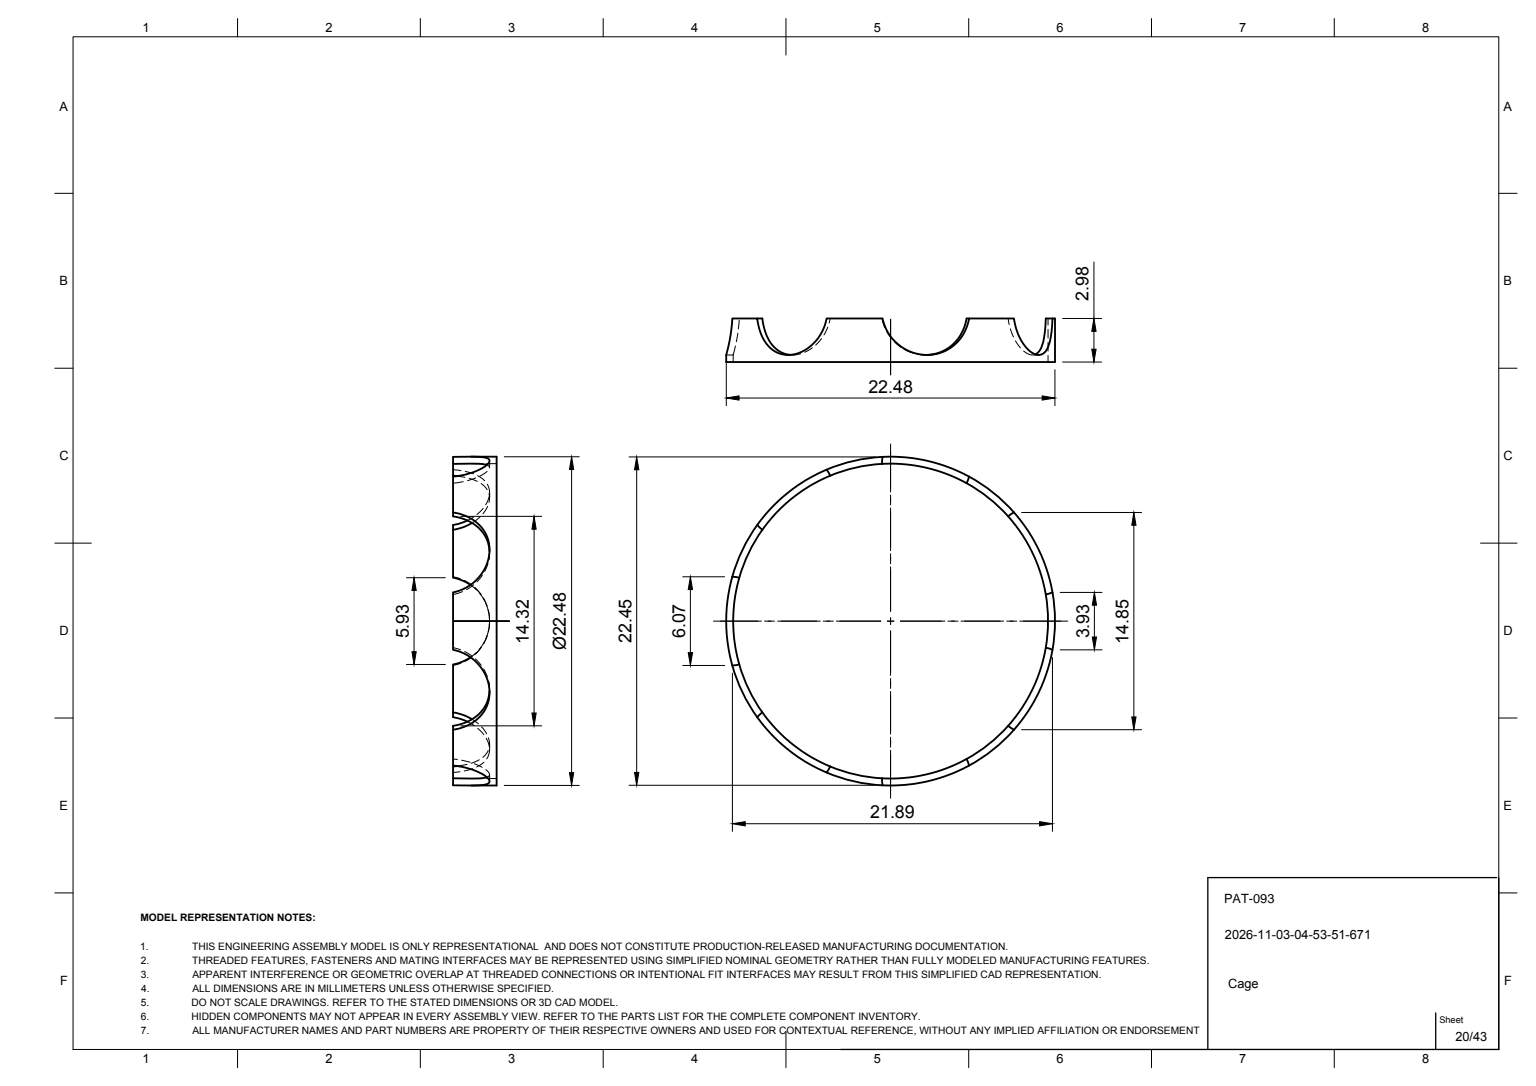
ISO-10303-21;
HEADER;
/* Generated by software containing ST-Developer
 * from STEP Tools, Inc. (www.steptools.com) 
 */

FILE_DESCRIPTION(
/* description */ ('Self-centering screw clamp'),
/* implementation_level */ '2;1');

FILE_NAME(
/* name */ 'Cage.step',
/* time_stamp */ '2026-10-28T03:25:31-07:00',
/* author */ (''),
/* organization */ (''),
/* preprocessor_version */ 'ST-DEVELOPER v20.2',
/* originating_system */ 'Autodesk Translation Framework v15.17.0.0',
/* authorisation */ '');

FILE_SCHEMA (('AUTOMOTIVE_DESIGN { 1 0 10303 214 3 1 1 }'));
ENDSEC;

DATA;
#10=MECHANICAL_DESIGN_GEOMETRIC_PRESENTATION_REPRESENTATION('',(#647),#16799);
#474=SPHERICAL_SURFACE('',#10011,0.309556);
#475=SPHERICAL_SURFACE('',#10027,0.309556);
#476=SPHERICAL_SURFACE('',#10032,0.309556);
#477=SPHERICAL_SURFACE('',#10038,0.309556);
#478=SPHERICAL_SURFACE('',#10043,0.309556);
#479=SPHERICAL_SURFACE('',#10048,0.309556);
#480=SPHERICAL_SURFACE('',#10056,0.309556);
#514=B_SPLINE_CURVE_WITH_KNOTS('',3,(#14785,#14786,#14787,#14788,#14789,
#14790,#14791,#14792,#14793,#14794,#14795,#14796,#14797,#14798,#14799,#14800,
#14801,#14802,#14803,#14804,#14805,#14806),.UNSPECIFIED.,.F.,.F.,(4,2,2,
2,2,2,2,2,2,2,4),(0.0591825211272536,0.157966726598481,0.236950089897721,
0.315933453196962,0.391576304923761,0.46721915665056,0.54286200837736,0.618504860104159,
0.697488223403399,0.77647158670264,0.875255792173867),.UNSPECIFIED.);
#515=B_SPLINE_CURVE_WITH_KNOTS('',3,(#14810,#14811,#14812,#14813,#14814,
#14815,#14816,#14817,#14818,#14819,#14820,#14821,#14822,#14823,#14824,#14825,
#14826,#14827,#14828,#14829,#14830,#14831),.UNSPECIFIED.,.F.,.F.,(4,2,2,
2,2,2,2,2,2,2,4),(0.0581119756758434,0.106553146291161,0.213106292582322,
0.30849933801665,0.386091982889075,0.4636846277615,0.541277272633925,0.61886991750635,
0.714262962940678,0.820816109231839,0.869257279847157),.UNSPECIFIED.);
#516=B_SPLINE_CURVE_WITH_KNOTS('',3,(#14837,#14838,#14839,#14840,#14841,
#14842,#14843,#14844,#14845,#14846,#14847,#14848,#14849,#14850,#14851,#14852,
#14853,#14854,#14855,#14856,#14857,#14858),.UNSPECIFIED.,.F.,.F.,(4,2,2,
2,2,2,2,2,2,2,4),(0.0581119756758434,0.106553146291161,0.213106292582322,
0.30849933801665,0.386091982889075,0.4636846277615,0.541277272633925,0.61886991750635,
0.714262962940679,0.820816109231839,0.869257279847157),.UNSPECIFIED.);
#517=B_SPLINE_CURVE_WITH_KNOTS('',3,(#14862,#14863,#14864,#14865,#14866,
#14867,#14868,#14869,#14870,#14871,#14872,#14873,#14874,#14875,#14876,#14877,
#14878,#14879,#14880,#14881,#14882,#14883),.UNSPECIFIED.,.F.,.F.,(4,2,2,
2,2,2,2,2,2,2,4),(0.0581119756758433,0.106553146291161,0.213106292582322,
0.308499338016649,0.386091982889075,0.4636846277615,0.541277272633925,0.61886991750635,
0.714262962940678,0.820816109231839,0.869257279847157),.UNSPECIFIED.);
#518=B_SPLINE_CURVE_WITH_KNOTS('',3,(#14892,#14893,#14894,#14895,#14896,
#14897,#14898,#14899,#14900,#14901,#14902,#14903,#14904,#14905,#14906,#14907,
#14908,#14909,#14910,#14911,#14912,#14913),.UNSPECIFIED.,.F.,.F.,(4,2,2,
2,2,2,2,2,2,2,4),(0.0581119756758433,0.106553146291161,0.213106292582322,
0.30849933801665,0.386091982889075,0.4636846277615,0.541277272633925,0.61886991750635,
0.714262962940678,0.820816109231839,0.869257279847157),.UNSPECIFIED.);
#519=B_SPLINE_CURVE_WITH_KNOTS('',3,(#14917,#14918,#14919,#14920,#14921,
#14922,#14923,#14924,#14925,#14926,#14927,#14928,#14929,#14930,#14931,#14932,
#14933,#14934,#14935,#14936,#14937,#14938),.UNSPECIFIED.,.F.,.F.,(4,2,2,
2,2,2,2,2,2,2,4),(0.0581119756758434,0.106553146291161,0.213106292582322,
0.30849933801665,0.386091982889075,0.4636846277615,0.541277272633925,0.61886991750635,
0.714262962940678,0.820816109231839,0.869257279847157),.UNSPECIFIED.);
#520=B_SPLINE_CURVE_WITH_KNOTS('',3,(#14942,#14943,#14944,#14945,#14946,
#14947,#14948,#14949,#14950,#14951,#14952,#14953,#14954,#14955,#14956,#14957,
#14958,#14959,#14960,#14961,#14962,#14963),.UNSPECIFIED.,.F.,.F.,(4,2,2,
2,2,2,2,2,2,2,4),(0.0581119756758434,0.106553146291161,0.213106292582322,
0.30849933801665,0.386091982889075,0.4636846277615,0.541277272633925,0.61886991750635,
0.714262962940678,0.820816109231839,0.869257279847157),.UNSPECIFIED.);
#521=B_SPLINE_CURVE_WITH_KNOTS('',3,(#14967,#14968,#14969,#14970,#14971,
#14972,#14973,#14974,#14975,#14976,#14977,#14978,#14979,#14980,#14981,#14982,
#14983,#14984,#14985,#14986,#14987,#14988),.UNSPECIFIED.,.F.,.F.,(4,2,2,
2,2,2,2,2,2,2,4),(0.0581119756758433,0.106553146291161,0.213106292582322,
0.30849933801665,0.386091982889075,0.4636846277615,0.541277272633925,0.61886991750635,
0.714262962940678,0.820816109231839,0.869257279847157),.UNSPECIFIED.);
#522=B_SPLINE_CURVE_WITH_KNOTS('',3,(#14996,#14997,#14998,#14999,#15000,
#15001,#15002,#15003,#15004,#15005,#15006,#15007,#15008,#15009,#15010,#15011,
#15012,#15013,#15014,#15015,#15016,#15017),.UNSPECIFIED.,.F.,.F.,(4,2,2,
2,2,2,2,2,2,2,4),(0.0591825211272536,0.157966726598481,0.236950089897721,
0.315933453196962,0.391576304923761,0.467219156650561,0.54286200837736,
0.618504860104159,0.697488223403399,0.77647158670264,0.875255792173867),
 .UNSPECIFIED.);
#523=B_SPLINE_CURVE_WITH_KNOTS('',3,(#15025,#15026,#15027,#15028,#15029,
#15030,#15031,#15032,#15033,#15034,#15035,#15036,#15037,#15038,#15039,#15040,
#15041,#15042,#15043,#15044,#15045,#15046),.UNSPECIFIED.,.F.,.F.,(4,2,2,
2,2,2,2,2,2,2,4),(0.0591825211272536,0.157966726598481,0.236950089897722,
0.315933453196962,0.391576304923761,0.467219156650561,0.54286200837736,
0.618504860104159,0.697488223403399,0.77647158670264,0.875255792173867),
 .UNSPECIFIED.);
#524=B_SPLINE_CURVE_WITH_KNOTS('',3,(#15056,#15057,#15058,#15059,#15060,
#15061,#15062,#15063,#15064,#15065,#15066,#15067,#15068,#15069,#15070,#15071,
#15072,#15073,#15074,#15075,#15076,#15077),.UNSPECIFIED.,.F.,.F.,(4,2,2,
2,2,2,2,2,2,2,4),(0.0591825211272536,0.157966726598481,0.236950089897721,
0.315933453196962,0.391576304923761,0.46721915665056,0.54286200837736,0.618504860104159,
0.697488223403399,0.77647158670264,0.875255792173867),.UNSPECIFIED.);
#525=B_SPLINE_CURVE_WITH_KNOTS('',3,(#15085,#15086,#15087,#15088,#15089,
#15090,#15091,#15092,#15093,#15094,#15095,#15096,#15097,#15098,#15099,#15100,
#15101,#15102,#15103,#15104,#15105,#15106),.UNSPECIFIED.,.F.,.F.,(4,2,2,
2,2,2,2,2,2,2,4),(0.0591825211272536,0.157966726598481,0.236950089897721,
0.315933453196962,0.391576304923761,0.46721915665056,0.542862008377359,
0.618504860104159,0.697488223403399,0.776471586702639,0.875255792173867),
 .UNSPECIFIED.);
#526=B_SPLINE_CURVE_WITH_KNOTS('',3,(#15114,#15115,#15116,#15117,#15118,
#15119,#15120,#15121,#15122,#15123,#15124,#15125,#15126,#15127,#15128,#15129,
#15130,#15131,#15132,#15133,#15134,#15135),.UNSPECIFIED.,.F.,.F.,(4,2,2,
2,2,2,2,2,2,2,4),(0.0591825211272536,0.157966726598481,0.236950089897721,
0.315933453196962,0.391576304923761,0.46721915665056,0.54286200837736,0.618504860104159,
0.697488223403399,0.77647158670264,0.875255792173867),.UNSPECIFIED.);
#527=B_SPLINE_CURVE_WITH_KNOTS('',3,(#15144,#15145,#15146,#15147,#15148,
#15149,#15150,#15151,#15152,#15153,#15154,#15155,#15156,#15157,#15158,#15159,
#15160,#15161,#15162,#15163,#15164,#15165),.UNSPECIFIED.,.F.,.F.,(4,2,2,
2,2,2,2,2,2,2,4),(0.0591825211272536,0.157966726598481,0.236950089897721,
0.315933453196962,0.391576304923761,0.46721915665056,0.542862008377359,
0.618504860104159,0.697488223403399,0.776471586702639,0.875255792173867),
 .UNSPECIFIED.);
#559=SHAPE_REPRESENTATION_RELATIONSHIP('SRR','None',#17033,#600);
#600=ADVANCED_BREP_SHAPE_REPRESENTATION('',(#695),#16771);
#647=STYLED_ITEM('',(#17326),#695);
#695=MANIFOLD_SOLID_BREP('Continuous crown cage',#9098);
#846=FACE_BOUND('',#2125,.T.);
#1110=PLANE('',#10024);
#1111=PLANE('',#10029);
#1112=PLANE('',#10034);
#1113=PLANE('',#10040);
#1114=PLANE('',#10045);
#1115=PLANE('',#10054);
#1116=PLANE('',#10058);
#1117=PLANE('',#10059);
#1477=FACE_OUTER_BOUND('',#2109,.T.);
#1478=FACE_OUTER_BOUND('',#2110,.T.);
#1479=FACE_OUTER_BOUND('',#2111,.T.);
#1480=FACE_OUTER_BOUND('',#2112,.T.);
#1481=FACE_OUTER_BOUND('',#2113,.T.);
#1482=FACE_OUTER_BOUND('',#2114,.T.);
#1483=FACE_OUTER_BOUND('',#2115,.T.);
#1484=FACE_OUTER_BOUND('',#2116,.T.);
#1485=FACE_OUTER_BOUND('',#2117,.T.);
#1486=FACE_OUTER_BOUND('',#2118,.T.);
#1487=FACE_OUTER_BOUND('',#2119,.T.);
#1488=FACE_OUTER_BOUND('',#2120,.T.);
#1489=FACE_OUTER_BOUND('',#2121,.T.);
#1490=FACE_OUTER_BOUND('',#2122,.T.);
#1491=FACE_OUTER_BOUND('',#2123,.T.);
#1492=FACE_OUTER_BOUND('',#2124,.T.);
#1493=FACE_OUTER_BOUND('',#2126,.T.);
#2109=EDGE_LOOP('',(#7071,#7072,#7073,#7074));
#2110=EDGE_LOOP('',(#7075,#7076,#7077,#7078,#7079,#7080,#7081,#7082,#7083,
#7084,#7085,#7086,#7087,#7088,#7089,#7090,#7091,#7092));
#2111=EDGE_LOOP('',(#7093,#7094,#7095,#7096));
#2112=EDGE_LOOP('',(#7097,#7098,#7099,#7100));
#2113=EDGE_LOOP('',(#7101,#7102,#7103,#7104));
#2114=EDGE_LOOP('',(#7105,#7106,#7107,#7108));
#2115=EDGE_LOOP('',(#7109,#7110,#7111,#7112,#7113,#7114));
#2116=EDGE_LOOP('',(#7115,#7116,#7117,#7118));
#2117=EDGE_LOOP('',(#7119,#7120,#7121,#7122));
#2118=EDGE_LOOP('',(#7123,#7124,#7125,#7126));
#2119=EDGE_LOOP('',(#7127,#7128,#7129,#7130));
#2120=EDGE_LOOP('',(#7131,#7132,#7133,#7134));
#2121=EDGE_LOOP('',(#7135,#7136,#7137,#7138,#7139,#7140,#7141,#7142,#7143,
#7144,#7145,#7146,#7147,#7148,#7149,#7150,#7151,#7152));
#2122=EDGE_LOOP('',(#7153,#7154,#7155,#7156));
#2123=EDGE_LOOP('',(#7157,#7158,#7159,#7160));
#2124=EDGE_LOOP('',(#7161));
#2125=EDGE_LOOP('',(#7162));
#2126=EDGE_LOOP('',(#7163,#7164,#7165,#7166));
#2836=LINE('',#14887,#3409);
#2837=LINE('',#15140,#3410);
#3409=VECTOR('',#11893,1.123812);
#3410=VECTOR('',#11962,1.076188);
#3932=CIRCLE('',#10012,0.303778037777585);
#3933=CIRCLE('',#10013,0.303778037777585);
#3934=CIRCLE('',#10015,1.123812);
#3935=CIRCLE('',#10016,1.123812);
#3936=CIRCLE('',#10017,1.123812);
#3937=CIRCLE('',#10018,1.123812);
#3938=CIRCLE('',#10019,1.123812);
#3939=CIRCLE('',#10020,1.123812);
#3940=CIRCLE('',#10021,1.123812);
#3941=CIRCLE('',#10022,1.123812);
#3942=CIRCLE('',#10023,1.123812);
#3943=CIRCLE('',#10025,1.076188);
#3944=CIRCLE('',#10026,0.303778037777585);
#3945=CIRCLE('',#10028,0.303778037777585);
#3946=CIRCLE('',#10030,1.076188);
#3947=CIRCLE('',#10031,0.303778037777585);
#3948=CIRCLE('',#10033,0.303778037777585);
#3949=CIRCLE('',#10035,1.076188);
#3950=CIRCLE('',#10036,1.076188);
#3951=CIRCLE('',#10037,0.303778037777585);
#3952=CIRCLE('',#10039,0.303778037777585);
#3953=CIRCLE('',#10041,1.076188);
#3954=CIRCLE('',#10042,0.303778037777585);
#3955=CIRCLE('',#10044,0.303778037777585);
#3956=CIRCLE('',#10046,1.076188);
#3957=CIRCLE('',#10047,0.303778037777585);
#3958=CIRCLE('',#10049,0.303778037777585);
#3959=CIRCLE('',#10051,1.076188);
#3960=CIRCLE('',#10052,1.076188);
#3961=CIRCLE('',#10053,1.076188);
#3962=CIRCLE('',#10055,0.303778037777585);
#3963=CIRCLE('',#10057,0.303778037777585);
#4551=VERTEX_POINT('',#14783);
#4552=VERTEX_POINT('',#14784);
#4553=VERTEX_POINT('',#14807);
#4554=VERTEX_POINT('',#14809);
#4555=VERTEX_POINT('',#14834);
#4556=VERTEX_POINT('',#14836);
#4557=VERTEX_POINT('',#14859);
#4558=VERTEX_POINT('',#14861);
#4559=VERTEX_POINT('',#14884);
#4560=VERTEX_POINT('',#14886);
#4561=VERTEX_POINT('',#14889);
#4562=VERTEX_POINT('',#14891);
#4563=VERTEX_POINT('',#14914);
#4564=VERTEX_POINT('',#14916);
#4565=VERTEX_POINT('',#14939);
#4566=VERTEX_POINT('',#14941);
#4567=VERTEX_POINT('',#14964);
#4568=VERTEX_POINT('',#14966);
#4569=VERTEX_POINT('',#14991);
#4570=VERTEX_POINT('',#14995);
#4571=VERTEX_POINT('',#15020);
#4572=VERTEX_POINT('',#15024);
#4573=VERTEX_POINT('',#15049);
#4574=VERTEX_POINT('',#15051);
#4575=VERTEX_POINT('',#15055);
#4576=VERTEX_POINT('',#15080);
#4577=VERTEX_POINT('',#15084);
#4578=VERTEX_POINT('',#15109);
#4579=VERTEX_POINT('',#15113);
#4580=VERTEX_POINT('',#15138);
#4581=VERTEX_POINT('',#15141);
#4582=VERTEX_POINT('',#15143);
#5460=EDGE_CURVE('',#4551,#4552,#514,.T.);
#5461=EDGE_CURVE('',#4553,#4551,#3932,.T.);
#5462=EDGE_CURVE('',#4554,#4553,#515,.T.);
#5463=EDGE_CURVE('',#4552,#4554,#3933,.T.);
#5464=EDGE_CURVE('',#4555,#4553,#3934,.T.);
#5465=EDGE_CURVE('',#4555,#4556,#516,.T.);
#5466=EDGE_CURVE('',#4557,#4556,#3935,.T.);
#5467=EDGE_CURVE('',#4557,#4558,#517,.T.);
#5468=EDGE_CURVE('',#4559,#4558,#3936,.T.);
#5469=EDGE_CURVE('',#4559,#4560,#2836,.T.);
#5470=EDGE_CURVE('',#4560,#4560,#3937,.T.);
#5471=EDGE_CURVE('',#4561,#4559,#3938,.T.);
#5472=EDGE_CURVE('',#4561,#4562,#518,.T.);
#5473=EDGE_CURVE('',#4563,#4562,#3939,.T.);
#5474=EDGE_CURVE('',#4563,#4564,#519,.T.);
#5475=EDGE_CURVE('',#4565,#4564,#3940,.T.);
#5476=EDGE_CURVE('',#4565,#4566,#520,.T.);
#5477=EDGE_CURVE('',#4567,#4566,#3941,.T.);
#5478=EDGE_CURVE('',#4567,#4568,#521,.T.);
#5479=EDGE_CURVE('',#4554,#4568,#3942,.T.);
#5480=EDGE_CURVE('',#4551,#4569,#3943,.T.);
#5481=EDGE_CURVE('',#4569,#4555,#3944,.T.);
#5482=EDGE_CURVE('',#4570,#4569,#522,.T.);
#5483=EDGE_CURVE('',#4556,#4570,#3945,.T.);
#5484=EDGE_CURVE('',#4570,#4571,#3946,.T.);
#5485=EDGE_CURVE('',#4571,#4557,#3947,.T.);
#5486=EDGE_CURVE('',#4572,#4571,#523,.T.);
#5487=EDGE_CURVE('',#4558,#4572,#3948,.T.);
#5488=EDGE_CURVE('',#4572,#4573,#3949,.T.);
#5489=EDGE_CURVE('',#4573,#4574,#3950,.T.);
#5490=EDGE_CURVE('',#4574,#4561,#3951,.T.);
#5491=EDGE_CURVE('',#4575,#4574,#524,.T.);
#5492=EDGE_CURVE('',#4562,#4575,#3952,.T.);
#5493=EDGE_CURVE('',#4575,#4576,#3953,.T.);
#5494=EDGE_CURVE('',#4576,#4563,#3954,.T.);
#5495=EDGE_CURVE('',#4577,#4576,#525,.T.);
#5496=EDGE_CURVE('',#4564,#4577,#3955,.T.);
#5497=EDGE_CURVE('',#4577,#4578,#3956,.T.);
#5498=EDGE_CURVE('',#4578,#4565,#3957,.T.);
#5499=EDGE_CURVE('',#4579,#4578,#526,.T.);
#5500=EDGE_CURVE('',#4566,#4579,#3958,.T.);
#5501=EDGE_CURVE('',#4580,#4580,#3959,.T.);
#5502=EDGE_CURVE('',#4580,#4573,#2837,.T.);
#5503=EDGE_CURVE('',#4581,#4552,#3960,.T.);
#5504=EDGE_CURVE('',#4581,#4582,#527,.T.);
#5505=EDGE_CURVE('',#4579,#4582,#3961,.T.);
#5506=EDGE_CURVE('',#4568,#4581,#3962,.T.);
#5507=EDGE_CURVE('',#4582,#4567,#3963,.T.);
#7071=ORIENTED_EDGE('',*,*,#5460,.F.);
#7072=ORIENTED_EDGE('',*,*,#5461,.F.);
#7073=ORIENTED_EDGE('',*,*,#5462,.F.);
#7074=ORIENTED_EDGE('',*,*,#5463,.F.);
#7075=ORIENTED_EDGE('',*,*,#5462,.T.);
#7076=ORIENTED_EDGE('',*,*,#5464,.F.);
#7077=ORIENTED_EDGE('',*,*,#5465,.T.);
#7078=ORIENTED_EDGE('',*,*,#5466,.F.);
#7079=ORIENTED_EDGE('',*,*,#5467,.T.);
#7080=ORIENTED_EDGE('',*,*,#5468,.F.);
#7081=ORIENTED_EDGE('',*,*,#5469,.T.);
#7082=ORIENTED_EDGE('',*,*,#5470,.F.);
#7083=ORIENTED_EDGE('',*,*,#5469,.F.);
#7084=ORIENTED_EDGE('',*,*,#5471,.F.);
#7085=ORIENTED_EDGE('',*,*,#5472,.T.);
#7086=ORIENTED_EDGE('',*,*,#5473,.F.);
#7087=ORIENTED_EDGE('',*,*,#5474,.T.);
#7088=ORIENTED_EDGE('',*,*,#5475,.F.);
#7089=ORIENTED_EDGE('',*,*,#5476,.T.);
#7090=ORIENTED_EDGE('',*,*,#5477,.F.);
#7091=ORIENTED_EDGE('',*,*,#5478,.T.);
#7092=ORIENTED_EDGE('',*,*,#5479,.F.);
#7093=ORIENTED_EDGE('',*,*,#5461,.T.);
#7094=ORIENTED_EDGE('',*,*,#5480,.T.);
#7095=ORIENTED_EDGE('',*,*,#5481,.T.);
#7096=ORIENTED_EDGE('',*,*,#5464,.T.);
#7097=ORIENTED_EDGE('',*,*,#5482,.F.);
#7098=ORIENTED_EDGE('',*,*,#5483,.F.);
#7099=ORIENTED_EDGE('',*,*,#5465,.F.);
#7100=ORIENTED_EDGE('',*,*,#5481,.F.);
#7101=ORIENTED_EDGE('',*,*,#5483,.T.);
#7102=ORIENTED_EDGE('',*,*,#5484,.T.);
#7103=ORIENTED_EDGE('',*,*,#5485,.T.);
#7104=ORIENTED_EDGE('',*,*,#5466,.T.);
#7105=ORIENTED_EDGE('',*,*,#5486,.F.);
#7106=ORIENTED_EDGE('',*,*,#5487,.F.);
#7107=ORIENTED_EDGE('',*,*,#5467,.F.);
#7108=ORIENTED_EDGE('',*,*,#5485,.F.);
#7109=ORIENTED_EDGE('',*,*,#5487,.T.);
#7110=ORIENTED_EDGE('',*,*,#5488,.T.);
#7111=ORIENTED_EDGE('',*,*,#5489,.T.);
#7112=ORIENTED_EDGE('',*,*,#5490,.T.);
#7113=ORIENTED_EDGE('',*,*,#5471,.T.);
#7114=ORIENTED_EDGE('',*,*,#5468,.T.);
#7115=ORIENTED_EDGE('',*,*,#5491,.F.);
#7116=ORIENTED_EDGE('',*,*,#5492,.F.);
#7117=ORIENTED_EDGE('',*,*,#5472,.F.);
#7118=ORIENTED_EDGE('',*,*,#5490,.F.);
#7119=ORIENTED_EDGE('',*,*,#5492,.T.);
#7120=ORIENTED_EDGE('',*,*,#5493,.T.);
#7121=ORIENTED_EDGE('',*,*,#5494,.T.);
#7122=ORIENTED_EDGE('',*,*,#5473,.T.);
#7123=ORIENTED_EDGE('',*,*,#5495,.F.);
#7124=ORIENTED_EDGE('',*,*,#5496,.F.);
#7125=ORIENTED_EDGE('',*,*,#5474,.F.);
#7126=ORIENTED_EDGE('',*,*,#5494,.F.);
#7127=ORIENTED_EDGE('',*,*,#5496,.T.);
#7128=ORIENTED_EDGE('',*,*,#5497,.T.);
#7129=ORIENTED_EDGE('',*,*,#5498,.T.);
#7130=ORIENTED_EDGE('',*,*,#5475,.T.);
#7131=ORIENTED_EDGE('',*,*,#5476,.F.);
#7132=ORIENTED_EDGE('',*,*,#5498,.F.);
#7133=ORIENTED_EDGE('',*,*,#5499,.F.);
#7134=ORIENTED_EDGE('',*,*,#5500,.F.);
#7135=ORIENTED_EDGE('',*,*,#5501,.F.);
#7136=ORIENTED_EDGE('',*,*,#5502,.T.);
#7137=ORIENTED_EDGE('',*,*,#5488,.F.);
#7138=ORIENTED_EDGE('',*,*,#5486,.T.);
#7139=ORIENTED_EDGE('',*,*,#5484,.F.);
#7140=ORIENTED_EDGE('',*,*,#5482,.T.);
#7141=ORIENTED_EDGE('',*,*,#5480,.F.);
#7142=ORIENTED_EDGE('',*,*,#5460,.T.);
#7143=ORIENTED_EDGE('',*,*,#5503,.F.);
#7144=ORIENTED_EDGE('',*,*,#5504,.T.);
#7145=ORIENTED_EDGE('',*,*,#5505,.F.);
#7146=ORIENTED_EDGE('',*,*,#5499,.T.);
#7147=ORIENTED_EDGE('',*,*,#5497,.F.);
#7148=ORIENTED_EDGE('',*,*,#5495,.T.);
#7149=ORIENTED_EDGE('',*,*,#5493,.F.);
#7150=ORIENTED_EDGE('',*,*,#5491,.T.);
#7151=ORIENTED_EDGE('',*,*,#5489,.F.);
#7152=ORIENTED_EDGE('',*,*,#5502,.F.);
#7153=ORIENTED_EDGE('',*,*,#5463,.T.);
#7154=ORIENTED_EDGE('',*,*,#5479,.T.);
#7155=ORIENTED_EDGE('',*,*,#5506,.T.);
#7156=ORIENTED_EDGE('',*,*,#5503,.T.);
#7157=ORIENTED_EDGE('',*,*,#5478,.F.);
#7158=ORIENTED_EDGE('',*,*,#5507,.F.);
#7159=ORIENTED_EDGE('',*,*,#5504,.F.);
#7160=ORIENTED_EDGE('',*,*,#5506,.F.);
#7161=ORIENTED_EDGE('',*,*,#5470,.T.);
#7162=ORIENTED_EDGE('',*,*,#5501,.T.);
#7163=ORIENTED_EDGE('',*,*,#5500,.T.);
#7164=ORIENTED_EDGE('',*,*,#5505,.T.);
#7165=ORIENTED_EDGE('',*,*,#5507,.T.);
#7166=ORIENTED_EDGE('',*,*,#5477,.T.);
#8450=CYLINDRICAL_SURFACE('',#10014,1.123812);
#8451=CYLINDRICAL_SURFACE('',#10050,1.076188);
#8775=ADVANCED_FACE('',(#1477),#474,.F.);
#8776=ADVANCED_FACE('',(#1478),#8450,.T.);
#8777=ADVANCED_FACE('',(#1479),#1110,.T.);
#8778=ADVANCED_FACE('',(#1480),#475,.F.);
#8779=ADVANCED_FACE('',(#1481),#1111,.T.);
#8780=ADVANCED_FACE('',(#1482),#476,.F.);
#8781=ADVANCED_FACE('',(#1483),#1112,.T.);
#8782=ADVANCED_FACE('',(#1484),#477,.F.);
#8783=ADVANCED_FACE('',(#1485),#1113,.T.);
#8784=ADVANCED_FACE('',(#1486),#478,.F.);
#8785=ADVANCED_FACE('',(#1487),#1114,.T.);
#8786=ADVANCED_FACE('',(#1488),#479,.F.);
#8787=ADVANCED_FACE('',(#1489),#8451,.F.);
#8788=ADVANCED_FACE('',(#1490),#1115,.T.);
#8789=ADVANCED_FACE('',(#1491),#480,.F.);
#8790=ADVANCED_FACE('',(#1492,#846),#1116,.T.);
#8791=ADVANCED_FACE('',(#1493),#1117,.T.);
#9098=CLOSED_SHELL('',(#8775,#8776,#8777,#8778,#8779,#8780,#8781,#8782,
#8783,#8784,#8785,#8786,#8787,#8788,#8789,#8790,#8791));
#10010=AXIS2_PLACEMENT_3D('',#14781,#11877,#11878);
#10011=AXIS2_PLACEMENT_3D('',#14782,#11879,#11880);
#10012=AXIS2_PLACEMENT_3D('',#14808,#11881,#11882);
#10013=AXIS2_PLACEMENT_3D('',#14832,#11883,#11884);
#10014=AXIS2_PLACEMENT_3D('',#14833,#11885,#11886);
#10015=AXIS2_PLACEMENT_3D('',#14835,#11887,#11888);
#10016=AXIS2_PLACEMENT_3D('',#14860,#11889,#11890);
#10017=AXIS2_PLACEMENT_3D('',#14885,#11891,#11892);
#10018=AXIS2_PLACEMENT_3D('',#14888,#11894,#11895);
#10019=AXIS2_PLACEMENT_3D('',#14890,#11896,#11897);
#10020=AXIS2_PLACEMENT_3D('',#14915,#11898,#11899);
#10021=AXIS2_PLACEMENT_3D('',#14940,#11900,#11901);
#10022=AXIS2_PLACEMENT_3D('',#14965,#11902,#11903);
#10023=AXIS2_PLACEMENT_3D('',#14989,#11904,#11905);
#10024=AXIS2_PLACEMENT_3D('',#14990,#11906,#11907);
#10025=AXIS2_PLACEMENT_3D('',#14992,#11908,#11909);
#10026=AXIS2_PLACEMENT_3D('',#14993,#11910,#11911);
#10027=AXIS2_PLACEMENT_3D('',#14994,#11912,#11913);
#10028=AXIS2_PLACEMENT_3D('',#15018,#11914,#11915);
#10029=AXIS2_PLACEMENT_3D('',#15019,#11916,#11917);
#10030=AXIS2_PLACEMENT_3D('',#15021,#11918,#11919);
#10031=AXIS2_PLACEMENT_3D('',#15022,#11920,#11921);
#10032=AXIS2_PLACEMENT_3D('',#15023,#11922,#11923);
#10033=AXIS2_PLACEMENT_3D('',#15047,#11924,#11925);
#10034=AXIS2_PLACEMENT_3D('',#15048,#11926,#11927);
#10035=AXIS2_PLACEMENT_3D('',#15050,#11928,#11929);
#10036=AXIS2_PLACEMENT_3D('',#15052,#11930,#11931);
#10037=AXIS2_PLACEMENT_3D('',#15053,#11932,#11933);
#10038=AXIS2_PLACEMENT_3D('',#15054,#11934,#11935);
#10039=AXIS2_PLACEMENT_3D('',#15078,#11936,#11937);
#10040=AXIS2_PLACEMENT_3D('',#15079,#11938,#11939);
#10041=AXIS2_PLACEMENT_3D('',#15081,#11940,#11941);
#10042=AXIS2_PLACEMENT_3D('',#15082,#11942,#11943);
#10043=AXIS2_PLACEMENT_3D('',#15083,#11944,#11945);
#10044=AXIS2_PLACEMENT_3D('',#15107,#11946,#11947);
#10045=AXIS2_PLACEMENT_3D('',#15108,#11948,#11949);
#10046=AXIS2_PLACEMENT_3D('',#15110,#11950,#11951);
#10047=AXIS2_PLACEMENT_3D('',#15111,#11952,#11953);
#10048=AXIS2_PLACEMENT_3D('',#15112,#11954,#11955);
#10049=AXIS2_PLACEMENT_3D('',#15136,#11956,#11957);
#10050=AXIS2_PLACEMENT_3D('',#15137,#11958,#11959);
#10051=AXIS2_PLACEMENT_3D('',#15139,#11960,#11961);
#10052=AXIS2_PLACEMENT_3D('',#15142,#11963,#11964);
#10053=AXIS2_PLACEMENT_3D('',#15166,#11965,#11966);
#10054=AXIS2_PLACEMENT_3D('',#15167,#11967,#11968);
#10055=AXIS2_PLACEMENT_3D('',#15168,#11969,#11970);
#10056=AXIS2_PLACEMENT_3D('',#15169,#11971,#11972);
#10057=AXIS2_PLACEMENT_3D('',#15170,#11973,#11974);
#10058=AXIS2_PLACEMENT_3D('',#15171,#11975,#11976);
#10059=AXIS2_PLACEMENT_3D('',#15172,#11977,#11978);
#11877=DIRECTION('axis',(0.,0.,1.));
#11878=DIRECTION('refdir',(1.,0.,0.));
#11879=DIRECTION('center_axis',(0.,0.,1.));
#11880=DIRECTION('ref_axis',(1.,0.,0.));
#11881=DIRECTION('center_axis',(0.,-1.,0.));
#11882=DIRECTION('ref_axis',(0.,0.,-1.));
#11883=DIRECTION('center_axis',(0.,-1.,0.));
#11884=DIRECTION('ref_axis',(0.,0.,-1.));
#11885=DIRECTION('center_axis',(0.,1.,0.));
#11886=DIRECTION('ref_axis',(1.,0.,0.));
#11887=DIRECTION('center_axis',(0.,1.,0.));
#11888=DIRECTION('ref_axis',(1.,0.,0.));
#11889=DIRECTION('center_axis',(0.,1.,0.));
#11890=DIRECTION('ref_axis',(1.,0.,0.));
#11891=DIRECTION('center_axis',(0.,1.,0.));
#11892=DIRECTION('ref_axis',(1.,0.,0.));
#11893=DIRECTION('',(0.,-1.,0.));
#11894=DIRECTION('center_axis',(0.,-1.,0.));
#11895=DIRECTION('ref_axis',(1.,0.,0.));
#11896=DIRECTION('center_axis',(0.,1.,0.));
#11897=DIRECTION('ref_axis',(1.,0.,0.));
#11898=DIRECTION('center_axis',(0.,1.,0.));
#11899=DIRECTION('ref_axis',(1.,0.,0.));
#11900=DIRECTION('center_axis',(0.,1.,0.));
#11901=DIRECTION('ref_axis',(1.,0.,0.));
#11902=DIRECTION('center_axis',(0.,1.,0.));
#11903=DIRECTION('ref_axis',(1.,0.,0.));
#11904=DIRECTION('center_axis',(0.,1.,0.));
#11905=DIRECTION('ref_axis',(1.,0.,0.));
#11906=DIRECTION('center_axis',(0.,1.,0.));
#11907=DIRECTION('ref_axis',(1.,0.,0.));
#11908=DIRECTION('center_axis',(0.,-1.,0.));
#11909=DIRECTION('ref_axis',(1.,0.,0.));
#11910=DIRECTION('center_axis',(0.,-1.,0.));
#11911=DIRECTION('ref_axis',(0.,0.,-1.));
#11912=DIRECTION('center_axis',(8.96625347776458E-17,0.,1.));
#11913=DIRECTION('ref_axis',(1.,0.,0.));
#11914=DIRECTION('center_axis',(0.,-1.,0.));
#11915=DIRECTION('ref_axis',(0.,0.,-1.));
#11916=DIRECTION('center_axis',(0.,1.,0.));
#11917=DIRECTION('ref_axis',(1.,0.,0.));
#11918=DIRECTION('center_axis',(0.,-1.,0.));
#11919=DIRECTION('ref_axis',(1.,0.,0.));
#11920=DIRECTION('center_axis',(0.,-1.,0.));
#11921=DIRECTION('ref_axis',(0.,0.,-1.));
#11922=DIRECTION('center_axis',(0.,0.,1.));
#11923=DIRECTION('ref_axis',(1.,0.,0.));
#11924=DIRECTION('center_axis',(0.,-1.,0.));
#11925=DIRECTION('ref_axis',(0.,0.,-1.));
#11926=DIRECTION('center_axis',(0.,1.,0.));
#11927=DIRECTION('ref_axis',(1.,0.,0.));
#11928=DIRECTION('center_axis',(0.,-1.,0.));
#11929=DIRECTION('ref_axis',(1.,0.,0.));
#11930=DIRECTION('center_axis',(0.,-1.,0.));
#11931=DIRECTION('ref_axis',(1.,0.,0.));
#11932=DIRECTION('center_axis',(0.,-1.,0.));
#11933=DIRECTION('ref_axis',(0.,0.,-1.));
#11934=DIRECTION('center_axis',(0.,0.,1.));
#11935=DIRECTION('ref_axis',(1.,0.,0.));
#11936=DIRECTION('center_axis',(0.,-1.,0.));
#11937=DIRECTION('ref_axis',(0.,0.,-1.));
#11938=DIRECTION('center_axis',(0.,1.,0.));
#11939=DIRECTION('ref_axis',(1.,0.,0.));
#11940=DIRECTION('center_axis',(0.,-1.,0.));
#11941=DIRECTION('ref_axis',(1.,0.,0.));
#11942=DIRECTION('center_axis',(0.,-1.,0.));
#11943=DIRECTION('ref_axis',(0.,0.,-1.));
#11944=DIRECTION('center_axis',(8.96625347776458E-17,0.,1.));
#11945=DIRECTION('ref_axis',(1.,0.,0.));
#11946=DIRECTION('center_axis',(0.,-1.,0.));
#11947=DIRECTION('ref_axis',(0.,0.,-1.));
#11948=DIRECTION('center_axis',(0.,1.,0.));
#11949=DIRECTION('ref_axis',(1.,0.,0.));
#11950=DIRECTION('center_axis',(0.,-1.,0.));
#11951=DIRECTION('ref_axis',(1.,0.,0.));
#11952=DIRECTION('center_axis',(0.,-1.,0.));
#11953=DIRECTION('ref_axis',(0.,0.,-1.));
#11954=DIRECTION('center_axis',(0.,0.,1.));
#11955=DIRECTION('ref_axis',(1.,0.,0.));
#11956=DIRECTION('center_axis',(0.,-1.,0.));
#11957=DIRECTION('ref_axis',(0.,0.,-1.));
#11958=DIRECTION('center_axis',(0.,1.,0.));
#11959=DIRECTION('ref_axis',(1.,0.,0.));
#11960=DIRECTION('center_axis',(0.,1.,0.));
#11961=DIRECTION('ref_axis',(1.,0.,0.));
#11962=DIRECTION('',(0.,1.,0.));
#11963=DIRECTION('center_axis',(0.,-1.,0.));
#11964=DIRECTION('ref_axis',(1.,0.,0.));
#11965=DIRECTION('center_axis',(0.,-1.,0.));
#11966=DIRECTION('ref_axis',(1.,0.,0.));
#11967=DIRECTION('center_axis',(0.,1.,0.));
#11968=DIRECTION('ref_axis',(1.,0.,0.));
#11969=DIRECTION('center_axis',(0.,-1.,0.));
#11970=DIRECTION('ref_axis',(0.,0.,-1.));
#11971=DIRECTION('center_axis',(0.,0.,1.));
#11972=DIRECTION('ref_axis',(1.,0.,0.));
#11973=DIRECTION('center_axis',(0.,-1.,0.));
#11974=DIRECTION('ref_axis',(0.,0.,-1.));
#11975=DIRECTION('center_axis',(0.,-1.,0.));
#11976=DIRECTION('ref_axis',(-1.,0.,0.));
#11977=DIRECTION('center_axis',(0.,1.,0.));
#11978=DIRECTION('ref_axis',(1.,0.,0.));
#14781=CARTESIAN_POINT('',(0.,0.,0.));
#14782=CARTESIAN_POINT('Origin',(0.685838782044607,0.,0.860014630714833));
#14783=CARTESIAN_POINT('',(0.413083465285518,-0.05953,0.993751811093549));
#14784=CARTESIAN_POINT('',(0.876916659919095,-0.05953,0.623857181492959));
#14785=CARTESIAN_POINT('Ctrl Pts',(0.413083465285518,-0.05953,0.993751811093549));
#14786=CARTESIAN_POINT('Ctrl Pts',(0.419070565453383,-0.0925528133349865,
0.991263089003441));
#14787=CARTESIAN_POINT('Ctrl Pts',(0.430199341854858,-0.124911173756694,
0.986608710139579));
#14788=CARTESIAN_POINT('Ctrl Pts',(0.457978755888596,-0.177924977804098,
0.973971221090534));
#14789=CARTESIAN_POINT('Ctrl Pts',(0.473077587363685,-0.199697230012983,
0.966820759530997));
#14790=CARTESIAN_POINT('Ctrl Pts',(0.507057380724533,-0.237895043532788,
0.949440676105255));
#14791=CARTESIAN_POINT('Ctrl Pts',(0.525933334162555,-0.254319232363049,
0.939198248544428));
#14792=CARTESIAN_POINT('Ctrl Pts',(0.564362943424238,-0.28018331644634,
0.916597376014514));
#14793=CARTESIAN_POINT('Ctrl Pts',(0.585840553788742,-0.29104845371857,
0.903141581680914));
#14794=CARTESIAN_POINT('Ctrl Pts',(0.629305439856167,-0.30527573347708,
0.873412008702649));
#14795=CARTESIAN_POINT('Ctrl Pts',(0.651278921914856,-0.308638795020976,
0.857118508332695));
#14796=CARTESIAN_POINT('Ctrl Pts',(0.690705563850638,-0.308638795020976,
0.825676810575914));
#14797=CARTESIAN_POINT('Ctrl Pts',(0.711480111898423,-0.30527573347708,
0.807879894508811));
#14798=CARTESIAN_POINT('Ctrl Pts',(0.750136149454208,-0.29104845371857,
0.772120216227122));
#14799=CARTESIAN_POINT('Ctrl Pts',(0.768033796848072,-0.28018331644634,
0.754175290318038));
#14800=CARTESIAN_POINT('Ctrl Pts',(0.798619410861634,-0.254319232363049,
0.721738358858166));
#14801=CARTESIAN_POINT('Ctrl Pts',(0.812805334167529,-0.237895043532788,
0.705614819529209));
#14802=CARTESIAN_POINT('Ctrl Pts',(0.837310877969633,-0.199697230012983,
0.676354402927683));
#14803=CARTESIAN_POINT('Ctrl Pts',(0.847641868610495,-0.177924977804098,
0.663225258065736));
#14804=CARTESIAN_POINT('Ctrl Pts',(0.866144010579847,-0.124911173756694,
0.638954437806245));
#14805=CARTESIAN_POINT('Ctrl Pts',(0.873158080166742,-0.0925528133349865,
0.62914037979579));
#14806=CARTESIAN_POINT('Ctrl Pts',(0.876916659919095,-0.05953,0.623857181492959));
#14807=CARTESIAN_POINT('',(0.437601487681057,-0.05953,1.03511272300331));
#14808=CARTESIAN_POINT('Origin',(0.685838782044607,-0.05953,0.860014630714833));
#14809=CARTESIAN_POINT('',(0.911784794170997,-0.05953,0.656964154625313));
#14810=CARTESIAN_POINT('Ctrl Pts',(0.911784794170998,-0.0595300000000001,
0.656964154625312));
#14811=CARTESIAN_POINT('Ctrl Pts',(0.909827729890942,-0.0762225747374255,
0.659680317203144));
#14812=CARTESIAN_POINT('Ctrl Pts',(0.907004864562642,-0.0928409665394228,
0.663576540841106));
#14813=CARTESIAN_POINT('Ctrl Pts',(0.895234408667242,-0.144299303100741,
0.679480524217551));
#14814=CARTESIAN_POINT('Ctrl Pts',(0.882797231409153,-0.177024326825049,
0.695831250979106));
#14815=CARTESIAN_POINT('Ctrl Pts',(0.854332839576145,-0.227269801620064,
0.73042219438957));
#14816=CARTESIAN_POINT('Ctrl Pts',(0.834863020612702,-0.251265615809407,
0.752807465209441));
#14817=CARTESIAN_POINT('Ctrl Pts',(0.800439809856111,-0.279889827963178,
0.789147407129766));
#14818=CARTESIAN_POINT('Ctrl Pts',(0.781998747691871,-0.290879136862659,
0.80756613568454));
#14819=CARTESIAN_POINT('Ctrl Pts',(0.742239891936898,-0.305251990234487,
0.844254137480382));
#14820=CARTESIAN_POINT('Ctrl Pts',(0.720906778729541,-0.308638795020976,
0.862505527716294));
#14821=CARTESIAN_POINT('Ctrl Pts',(0.680463863683392,-0.308638795020976,
0.894757676234429));
#14822=CARTESIAN_POINT('Ctrl Pts',(0.657923009631182,-0.305251990234488,
0.91149460735272));
#14823=CARTESIAN_POINT('Ctrl Pts',(0.613307674922609,-0.290879136862659,
0.942092777160053));
#14824=CARTESIAN_POINT('Ctrl Pts',(0.591247219971725,-0.279889827963178,
0.955972930713954));
#14825=CARTESIAN_POINT('Ctrl Pts',(0.548158511259202,-0.251265615809407,
0.981446681891443));
#14826=CARTESIAN_POINT('Ctrl Pts',(0.522002043615455,-0.227269801620063,
0.995447160474328));
#14827=CARTESIAN_POINT('Ctrl Pts',(0.481944444320713,-0.177024326825049,
1.01550068154148));
#14828=CARTESIAN_POINT('Ctrl Pts',(0.463236132117164,-0.14429930310074,
1.0239876538093));
#14829=CARTESIAN_POINT('Ctrl Pts',(0.445111721969657,-0.0928409665394226,
1.03192403056628));
#14830=CARTESIAN_POINT('Ctrl Pts',(0.440685038163619,-0.0762225747374254,
1.03380912944435));
#14831=CARTESIAN_POINT('Ctrl Pts',(0.437601487681056,-0.05953,1.03511272300331));
#14832=CARTESIAN_POINT('Origin',(0.685838782044607,-0.05953,0.860014630714833));
#14833=CARTESIAN_POINT('Origin',(0.,-0.208355,0.));
#14834=CARTESIAN_POINT('',(0.0548532617164168,-0.05953,1.12247250791415));
#14835=CARTESIAN_POINT('Origin',(0.,-0.05953,0.));
#14836=CARTESIAN_POINT('',(-0.536443649899848,-0.05953,0.987512846410683));
#14837=CARTESIAN_POINT('Ctrl Pts',(0.0548532617164173,-0.0595300000000001,
1.12247250791414));
#14838=CARTESIAN_POINT('Ctrl Pts',(0.05150947068137,-0.0762225747374254,
1.12263591311425));
#14839=CARTESIAN_POINT('Ctrl Pts',(0.0467032526342597,-0.0928409665394227,
1.12285816383385));
#14840=CARTESIAN_POINT('Ctrl Pts',(0.0269302585198975,-0.144299303100741,
1.12357162229597));
#14841=CARTESIAN_POINT('Ctrl Pts',(0.006392292392153,-0.177024326825049,
1.12404235695137));
#14842=CARTESIAN_POINT('Ctrl Pts',(-0.0383992541984087,-0.227269801620063,
1.12335509974011));
#14843=CARTESIAN_POINT('Ctrl Pts',(-0.0680399972366993,-0.251265615809407,
1.12208997038458));
#14844=CARTESIAN_POINT('Ctrl Pts',(-0.117914228755037,-0.279889827963178,
1.1178344036749));
#14845=CARTESIAN_POINT('Ctrl Pts',(-0.14381238480104,-0.290879136862659,
1.11490049012186));
#14846=CARTESIAN_POINT('Ctrl Pts',(-0.19728546073067,-0.305251990234488,
1.10669035995599));
#14847=CARTESIAN_POINT('Ctrl Pts',(-0.224855950742601,-0.308638795020976,
1.10139101611326));
#14848=CARTESIAN_POINT('Ctrl Pts',(-0.275287440920027,-0.308638795020976,
1.0898803575765));
#14849=CARTESIAN_POINT('Ctrl Pts',(-0.302426893214945,-0.305251990234488,
1.08269251410343));
#14850=CARTESIAN_POINT('Ctrl Pts',(-0.35416671187353,-0.290879136862659,
1.06688848765783));
#14851=CARTESIAN_POINT('Ctrl Pts',(-0.3787731215897,-0.279889827963178,
1.05829506364875));
#14852=CARTESIAN_POINT('Ctrl Pts',(-0.425554672694338,-0.251265615809407,
1.04048957871266));
#14853=CARTESIAN_POINT('Ctrl Pts',(-0.452808978448581,-0.227269801620063,
1.02876878445619));
#14854=CARTESIAN_POINT('Ctrl Pts',(-0.493462957200432,-0.177024326825049,
1.0099536580922));
#14855=CARTESIAN_POINT('Ctrl Pts',(-0.511762781179148,-0.14429930310074,
1.00061845128527));
#14856=CARTESIAN_POINT('Ctrl Pts',(-0.529268075276157,-0.0928409665394226,
0.991396466802468));
#14857=CARTESIAN_POINT('Ctrl Pts',(-0.533501897135713,-0.0762225747374254,
0.989110885965947));
#14858=CARTESIAN_POINT('Ctrl Pts',(-0.536443649899848,-0.0595300000000001,
0.987512846410683));
#14859=CARTESIAN_POINT('',(-0.843383895613249,-0.05953,0.742736168477219));
#14860=CARTESIAN_POINT('Origin',(0.,-0.05953,0.));
#14861=CARTESIAN_POINT('',(-1.10653577764992,-0.05953,0.196295654879792));
#14862=CARTESIAN_POINT('Ctrl Pts',(-0.843383895613249,-0.0595300000000001,
0.742736168477219));
#14863=CARTESIAN_POINT('Ctrl Pts',(-0.84559647055299,-0.0762225747374255,
0.740223768851062));
#14864=CARTESIAN_POINT('Ctrl Pts',(-0.848766861100456,-0.0928409665394227,
0.736604687327351));
#14865=CARTESIAN_POINT('Ctrl Pts',(-0.861652925570091,-0.144299303100741,
0.721590372101268));
#14866=CARTESIAN_POINT('Ctrl Pts',(-0.87482617317514,-0.177024326825049,
0.705826641853758));
#14867=CARTESIAN_POINT('Ctrl Pts',(-0.902215926359523,-0.227269801620063,
0.670378702718353));
#14868=CARTESIAN_POINT('Ctrl Pts',(-0.919707509403859,-0.251265615809407,
0.646415841396062));
#14869=CARTESIAN_POINT('Ctrl Pts',(-0.947476448101718,-0.279889827963178,
0.604769294586516));
#14870=CARTESIAN_POINT('Ctrl Pts',(-0.961329858300736,-0.290879136862659,
0.582692035672022));
#14871=CARTESIAN_POINT('Ctrl Pts',(-0.988250837578047,-0.305251990234488,
0.535766169015486));
#14872=CARTESIAN_POINT('Ctrl Pts',(-1.00129756308006,-0.308638795020976,
0.510906605094603));
#14873=CARTESIAN_POINT('Ctrl Pts',(-1.02374168767024,-0.308638795020976,
0.46430090015576));
#14874=CARTESIAN_POINT('Ctrl Pts',(-1.03504317708586,-0.305251990234488,
0.438600874831839));
#14875=CARTESIAN_POINT('Ctrl Pts',(-1.05494634094458,-0.290879136862659,
0.388295406390235));
#14876=CARTESIAN_POINT('Ctrl Pts',(-1.06356957703048,-0.279889827963178,
0.363699428370917));
#14877=CARTESIAN_POINT('Ctrl Pts',(-1.0788165083757,-0.251265615809407,
0.316022600643821));
#14878=CARTESIAN_POINT('Ctrl Pts',(-1.08664560412098,-0.227269801620063,
0.287406530683752));
#14879=CARTESIAN_POINT('Ctrl Pts',(-1.09728268713976,-0.177024326825049,
0.243890930799337));
#14880=CARTESIAN_POINT('Ctrl Pts',(-1.10139388218929,-0.144299303100741,
0.22376314604679));
#14881=CARTESIAN_POINT('Ctrl Pts',(-1.10509821673782,-0.0928409665394227,
0.204327142733961));
#14882=CARTESIAN_POINT('Ctrl Pts',(-1.10595102243643,-0.0762225747374254,
0.199591971170104));
#14883=CARTESIAN_POINT('Ctrl Pts',(-1.10653577764992,-0.0595300000000001,
0.196295654879792));
#14884=CARTESIAN_POINT('',(-1.123812,-0.05953,1.37627276864339E-16));
#14885=CARTESIAN_POINT('Origin',(0.,-0.05953,0.));
#14886=CARTESIAN_POINT('',(-1.123812,-0.35718,1.37627276864339E-16));
#14887=CARTESIAN_POINT('',(-1.123812,-0.208355,1.37627276864339E-16));
#14888=CARTESIAN_POINT('Origin',(0.,-0.35718,0.));
#14889=CARTESIAN_POINT('',(-1.10653577764992,-0.05953,-0.196295654879793));
#14890=CARTESIAN_POINT('Origin',(0.,-0.05953,0.));
#14891=CARTESIAN_POINT('',(-0.843383895613249,-0.05953,-0.742736168477219));
#14892=CARTESIAN_POINT('Ctrl Pts',(-1.10653577764992,-0.0595300000000001,
-0.196295654879792));
#14893=CARTESIAN_POINT('Ctrl Pts',(-1.10595102243643,-0.0762225747374255,
-0.199591971170104));
#14894=CARTESIAN_POINT('Ctrl Pts',(-1.10509821673782,-0.0928409665394228,
-0.204327142733962));
#14895=CARTESIAN_POINT('Ctrl Pts',(-1.10139388218929,-0.144299303100741,
-0.22376314604679));
#14896=CARTESIAN_POINT('Ctrl Pts',(-1.09728268713976,-0.177024326825049,
-0.243890930799338));
#14897=CARTESIAN_POINT('Ctrl Pts',(-1.08664560412098,-0.227269801620063,
-0.287406530683753));
#14898=CARTESIAN_POINT('Ctrl Pts',(-1.0788165083757,-0.251265615809407,
-0.316022600643821));
#14899=CARTESIAN_POINT('Ctrl Pts',(-1.06356957703048,-0.279889827963178,
-0.363699428370918));
#14900=CARTESIAN_POINT('Ctrl Pts',(-1.05494634094458,-0.290879136862659,
-0.388295406390235));
#14901=CARTESIAN_POINT('Ctrl Pts',(-1.03504317708586,-0.305251990234488,
-0.438600874831839));
#14902=CARTESIAN_POINT('Ctrl Pts',(-1.02374168767024,-0.308638795020976,
-0.46430090015576));
#14903=CARTESIAN_POINT('Ctrl Pts',(-1.00129756308006,-0.308638795020976,
-0.510906605094603));
#14904=CARTESIAN_POINT('Ctrl Pts',(-0.988250837578047,-0.305251990234488,
-0.535766169015486));
#14905=CARTESIAN_POINT('Ctrl Pts',(-0.961329858300736,-0.290879136862659,
-0.582692035672022));
#14906=CARTESIAN_POINT('Ctrl Pts',(-0.947476448101718,-0.279889827963178,
-0.604769294586516));
#14907=CARTESIAN_POINT('Ctrl Pts',(-0.919707509403859,-0.251265615809407,
-0.646415841396062));
#14908=CARTESIAN_POINT('Ctrl Pts',(-0.902215926359523,-0.227269801620064,
-0.670378702718353));
#14909=CARTESIAN_POINT('Ctrl Pts',(-0.87482617317514,-0.177024326825049,
-0.705826641853758));
#14910=CARTESIAN_POINT('Ctrl Pts',(-0.861652925570091,-0.144299303100741,
-0.721590372101268));
#14911=CARTESIAN_POINT('Ctrl Pts',(-0.848766861100456,-0.0928409665394229,
-0.736604687327351));
#14912=CARTESIAN_POINT('Ctrl Pts',(-0.84559647055299,-0.0762225747374255,
-0.740223768851063));
#14913=CARTESIAN_POINT('Ctrl Pts',(-0.843383895613249,-0.0595300000000001,
-0.742736168477219));
#14914=CARTESIAN_POINT('',(-0.536443649899847,-0.05953,-0.987512846410683));
#14915=CARTESIAN_POINT('Origin',(0.,-0.05953,0.));
#14916=CARTESIAN_POINT('',(0.0548532617164172,-0.05953,-1.12247250791415));
#14917=CARTESIAN_POINT('Ctrl Pts',(-0.536443649899848,-0.0595300000000001,
-0.987512846410683));
#14918=CARTESIAN_POINT('Ctrl Pts',(-0.533501897135712,-0.0762225747374254,
-0.989110885965947));
#14919=CARTESIAN_POINT('Ctrl Pts',(-0.529268075276156,-0.0928409665394227,
-0.991396466802469));
#14920=CARTESIAN_POINT('Ctrl Pts',(-0.511762781179147,-0.144299303100741,
-1.00061845128527));
#14921=CARTESIAN_POINT('Ctrl Pts',(-0.493462957200432,-0.177024326825049,
-1.0099536580922));
#14922=CARTESIAN_POINT('Ctrl Pts',(-0.45280897844858,-0.227269801620063,
-1.02876878445619));
#14923=CARTESIAN_POINT('Ctrl Pts',(-0.425554672694337,-0.251265615809407,
-1.04048957871266));
#14924=CARTESIAN_POINT('Ctrl Pts',(-0.3787731215897,-0.279889827963178,
-1.05829506364875));
#14925=CARTESIAN_POINT('Ctrl Pts',(-0.354166711873529,-0.290879136862659,
-1.06688848765783));
#14926=CARTESIAN_POINT('Ctrl Pts',(-0.302426893214944,-0.305251990234488,
-1.08269251410343));
#14927=CARTESIAN_POINT('Ctrl Pts',(-0.275287440920027,-0.308638795020976,
-1.0898803575765));
#14928=CARTESIAN_POINT('Ctrl Pts',(-0.224855950742601,-0.308638795020976,
-1.10139101611326));
#14929=CARTESIAN_POINT('Ctrl Pts',(-0.19728546073067,-0.305251990234488,
-1.10669035995599));
#14930=CARTESIAN_POINT('Ctrl Pts',(-0.143812384801039,-0.290879136862659,
-1.11490049012186));
#14931=CARTESIAN_POINT('Ctrl Pts',(-0.117914228755037,-0.279889827963178,
-1.1178344036749));
#14932=CARTESIAN_POINT('Ctrl Pts',(-0.0680399972366989,-0.251265615809407,
-1.12208997038458));
#14933=CARTESIAN_POINT('Ctrl Pts',(-0.0383992541984084,-0.227269801620063,
-1.12335509974011));
#14934=CARTESIAN_POINT('Ctrl Pts',(0.00639229239215326,-0.177024326825049,
-1.12404235695137));
#14935=CARTESIAN_POINT('Ctrl Pts',(0.0269302585198977,-0.144299303100741,
-1.12357162229597));
#14936=CARTESIAN_POINT('Ctrl Pts',(0.04670325263426,-0.0928409665394228,
-1.12285816383385));
#14937=CARTESIAN_POINT('Ctrl Pts',(0.0515094706813703,-0.0762225747374255,
-1.12263591311425));
#14938=CARTESIAN_POINT('Ctrl Pts',(0.0548532617164176,-0.0595300000000001,
-1.12247250791414));
#14939=CARTESIAN_POINT('',(0.437601487681057,-0.05953,-1.03511272300331));
#14940=CARTESIAN_POINT('Origin',(0.,-0.05953,0.));
#14941=CARTESIAN_POINT('',(0.911784794170997,-0.05953,-0.656964154625313));
#14942=CARTESIAN_POINT('Ctrl Pts',(0.437601487681056,-0.0595300000000001,
-1.03511272300331));
#14943=CARTESIAN_POINT('Ctrl Pts',(0.440685038163619,-0.0762225747374255,
-1.03380912944435));
#14944=CARTESIAN_POINT('Ctrl Pts',(0.445111721969657,-0.0928409665394228,
-1.03192403056628));
#14945=CARTESIAN_POINT('Ctrl Pts',(0.463236132117164,-0.144299303100741,
-1.0239876538093));
#14946=CARTESIAN_POINT('Ctrl Pts',(0.481944444320713,-0.177024326825049,
-1.01550068154148));
#14947=CARTESIAN_POINT('Ctrl Pts',(0.522002043615455,-0.227269801620064,
-0.995447160474328));
#14948=CARTESIAN_POINT('Ctrl Pts',(0.548158511259203,-0.251265615809407,
-0.981446681891443));
#14949=CARTESIAN_POINT('Ctrl Pts',(0.591247219971725,-0.279889827963178,
-0.955972930713954));
#14950=CARTESIAN_POINT('Ctrl Pts',(0.613307674922609,-0.290879136862659,
-0.942092777160053));
#14951=CARTESIAN_POINT('Ctrl Pts',(0.657923009631182,-0.305251990234487,
-0.91149460735272));
#14952=CARTESIAN_POINT('Ctrl Pts',(0.680463863683393,-0.308638795020976,
-0.894757676234429));
#14953=CARTESIAN_POINT('Ctrl Pts',(0.720906778729542,-0.308638795020976,
-0.862505527716294));
#14954=CARTESIAN_POINT('Ctrl Pts',(0.742239891936899,-0.305251990234488,
-0.844254137480381));
#14955=CARTESIAN_POINT('Ctrl Pts',(0.781998747691872,-0.290879136862659,
-0.80756613568454));
#14956=CARTESIAN_POINT('Ctrl Pts',(0.800439809856112,-0.279889827963178,
-0.789147407129765));
#14957=CARTESIAN_POINT('Ctrl Pts',(0.834863020612702,-0.251265615809407,
-0.752807465209441));
#14958=CARTESIAN_POINT('Ctrl Pts',(0.854332839576145,-0.227269801620064,
-0.73042219438957));
#14959=CARTESIAN_POINT('Ctrl Pts',(0.882797231409153,-0.177024326825049,
-0.695831250979106));
#14960=CARTESIAN_POINT('Ctrl Pts',(0.895234408667242,-0.144299303100741,
-0.679480524217551));
#14961=CARTESIAN_POINT('Ctrl Pts',(0.907004864562642,-0.0928409665394228,
-0.663576540841106));
#14962=CARTESIAN_POINT('Ctrl Pts',(0.909827729890942,-0.0762225747374256,
-0.659680317203144));
#14963=CARTESIAN_POINT('Ctrl Pts',(0.911784794170998,-0.0595300000000001,
-0.656964154625312));
#14964=CARTESIAN_POINT('',(1.08212377959455,-0.05953,-0.303251606722892));
#14965=CARTESIAN_POINT('Origin',(0.,-0.05953,0.));
#14966=CARTESIAN_POINT('',(1.08212377959455,-0.05953,0.303251606722892));
#14967=CARTESIAN_POINT('Ctrl Pts',(1.08212377959455,-0.0595300000000001,
-0.303251606722892));
#14968=CARTESIAN_POINT('Ctrl Pts',(1.0830271513892,-0.0762225747374255,
-0.300028012588062));
#14969=CARTESIAN_POINT('Ctrl Pts',(1.08431331394788,-0.0928409665394228,
-0.2953917518996));
#14970=CARTESIAN_POINT('Ctrl Pts',(1.08940878963422,-0.144299303100741,
-0.276273267473431));
#14971=CARTESIAN_POINT('Ctrl Pts',(1.09443784939331,-0.177024326825049,
-0.256354979351213));
#14972=CARTESIAN_POINT('Ctrl Pts',(1.10373487993589,-0.227269801620064,
-0.212533521233765));
#14973=CARTESIAN_POINT('Ctrl Pts',(1.10909715583869,-0.251265615809407,
-0.183354415742157));
#14974=CARTESIAN_POINT('Ctrl Pts',(1.1160463456491,-0.279889827963178,-0.133783682657561));
#14975=CARTESIAN_POINT('Ctrl Pts',(1.11894887330541,-0.290879136862659,
-0.107881990270302));
#14976=CARTESIAN_POINT('Ctrl Pts',(1.12284346704144,-0.305251990234488,
-0.0539226701638766));
#14977=CARTESIAN_POINT('Ctrl Pts',(1.123812,-0.308638795020976,-0.025864214957475));
#14978=CARTESIAN_POINT('Ctrl Pts',(1.123812,-0.308638795020976,0.025864214957475));
#14979=CARTESIAN_POINT('Ctrl Pts',(1.12284346704144,-0.305251990234488,
0.0539226701638766));
#14980=CARTESIAN_POINT('Ctrl Pts',(1.11894887330541,-0.290879136862659,
0.107881990270302));
#14981=CARTESIAN_POINT('Ctrl Pts',(1.1160463456491,-0.279889827963178,0.133783682657561));
#14982=CARTESIAN_POINT('Ctrl Pts',(1.10909715583869,-0.251265615809407,
0.183354415742157));
#14983=CARTESIAN_POINT('Ctrl Pts',(1.10373487993589,-0.227269801620064,
0.212533521233765));
#14984=CARTESIAN_POINT('Ctrl Pts',(1.09443784939331,-0.177024326825049,
0.256354979351213));
#14985=CARTESIAN_POINT('Ctrl Pts',(1.08940878963422,-0.144299303100741,
0.276273267473431));
#14986=CARTESIAN_POINT('Ctrl Pts',(1.08431331394788,-0.0928409665394228,
0.2953917518996));
#14987=CARTESIAN_POINT('Ctrl Pts',(1.0830271513892,-0.0762225747374255,
0.300028012588062));
#14988=CARTESIAN_POINT('Ctrl Pts',(1.08212377959455,-0.0595300000000001,
0.303251606722892));
#14989=CARTESIAN_POINT('Origin',(0.,-0.05953,0.));
#14990=CARTESIAN_POINT('Origin',(0.,-0.05953,0.));
#14991=CARTESIAN_POINT('',(0.0589974094846122,-0.05953,1.07456964270265));
#14992=CARTESIAN_POINT('Origin',(0.,-0.05953,0.));
#14993=CARTESIAN_POINT('Origin',(-0.244773027351946,-0.05953,1.07242070340001));
#14994=CARTESIAN_POINT('Origin',(-0.244773027351946,0.,1.07242070340001));
#14995=CARTESIAN_POINT('',(-0.519393123750572,-0.05953,0.942555777842682));
#14996=CARTESIAN_POINT('Ctrl Pts',(-0.519393123750572,-0.05953,0.942555777842682));
#14997=CARTESIAN_POINT('Ctrl Pts',(-0.513714466572041,-0.0925528133349865,
0.945684988399766));
#14998=CARTESIAN_POINT('Ctrl Pts',(-0.503136848051455,-0.124911173756694,
0.951483858396181));
#14999=CARTESIAN_POINT('Ctrl Pts',(-0.47593627990192,-0.177924977804098,
0.965323333309091));
#15000=CARTESIAN_POINT('Ctrl Pts',(-0.460931856495794,-0.199697230012983,
0.972669835243841));
#15001=CARTESIAN_POINT('Ctrl Pts',(-0.426157505475872,-0.237895043532788,
0.988400002689705));
#15002=CARTESIAN_POINT('Ctrl Pts',(-0.406380688682952,-0.254319232363049,
0.996771768218699));
#15003=CARTESIAN_POINT('Ctrl Pts',(-0.364750145543744,-0.28018331644634,
1.01272583306292));
#15004=CARTESIAN_POINT('Ctrl Pts',(-0.340838910881557,-0.29104845371857,
1.02112815447116));
#15005=CARTESIAN_POINT('Ctrl Pts',(-0.290495481564827,-0.30527573347708,
1.036574285215));
#15006=CARTESIAN_POINT('Ctrl Pts',(-0.264056468041074,-0.308638795020976,
1.04359501395068));
#15007=CARTESIAN_POINT('Ctrl Pts',(-0.214892249704082,-0.308638795020976,
1.05481642595959));
#15008=CARTESIAN_POINT('Ctrl Pts',(-0.188025341585962,-0.30527573347708,
1.05996242598502));
#15009=CARTESIAN_POINT('Ctrl Pts',(-0.135965654106109,-0.29104845371857,
1.06788913840721));
#15010=CARTESIAN_POINT('Ctrl Pts',(-0.110776745452494,-0.28018331644634,
1.07069360430242));
#15011=CARTESIAN_POINT('Ctrl Pts',(-0.0663467128214646,-0.254319232363049,
1.07438230428002));
#15012=CARTESIAN_POINT('Ctrl Pts',(-0.0448960436540983,-0.237895043532788,
1.07542044338697));
#15013=CARTESIAN_POINT('Ctrl Pts',(-0.00674037211528124,-0.199697230012983,
1.07633607767727));
#15014=CARTESIAN_POINT('Ctrl Pts',(0.00996567398334777,-0.177924977804098,
1.07622728347683));
#15015=CARTESIAN_POINT('Ctrl Pts',(0.0404772621979741,-0.124911173756694,
1.07556023164702));
#15016=CARTESIAN_POINT('Ctrl Pts',(0.0525234025782719,-0.0925528133349865,
1.07492508698591));
#15017=CARTESIAN_POINT('Ctrl Pts',(0.0589974094846124,-0.05953,1.07456964270265));
#15018=CARTESIAN_POINT('Origin',(-0.244773027351946,-0.05953,1.07242070340001));
#15019=CARTESIAN_POINT('Origin',(0.,-0.05953,0.));
#15020=CARTESIAN_POINT('',(-0.803348093619616,-0.05953,0.716109245731214));
#15021=CARTESIAN_POINT('Origin',(0.,-0.05953,0.));
#15022=CARTESIAN_POINT('Origin',(-0.991065754692661,-0.05953,0.477272113029314));
#15023=CARTESIAN_POINT('Origin',(-0.991065754692661,0.,0.477272113029314));
#15024=CARTESIAN_POINT('',(-1.06075609691358,-0.05953,0.181596019242328));
#15025=CARTESIAN_POINT('Ctrl Pts',(-1.06075609691358,-0.05953,0.181596019242328));
#15026=CARTESIAN_POINT('Ctrl Pts',(-1.05966202740332,-0.0925528133349865,
0.187986803072856));
#15027=CARTESIAN_POINT('Ctrl Pts',(-1.05760072925372,-0.124911173756694,
0.199872254546857));
#15028=CARTESIAN_POINT('Ctrl Pts',(-1.05146158959546,-0.177924977804098,
0.22976728653846));
#15029=CARTESIAN_POINT('Ctrl Pts',(-1.04785021111757,-0.199697230012983,
0.246078686169301));
#15030=CARTESIAN_POINT('Ctrl Pts',(-1.03846709802406,-0.237895043532788,
0.283073967563097));
#15031=CARTESIAN_POINT('Ctrl Pts',(-1.03268176429485,-0.254319232363049,
0.303755815985685));
#15032=CARTESIAN_POINT('Ctrl Pts',(-1.01919893537026,-0.28018331644634,
0.346251081972725));
#15033=CARTESIAN_POINT('Ctrl Pts',(-1.01085972381132,-0.29104845371857,
0.370184399726282));
#15034=CARTESIAN_POINT('Ctrl Pts',(-0.99154738033959,-0.30527573347708,
0.419174982698463));
#15035=CARTESIAN_POINT('Ctrl Pts',(-0.980551951791748,-0.308638795020976,
0.444223188605045));
#15036=CARTESIAN_POINT('Ctrl Pts',(-0.958671816228589,-0.308638795020976,
0.489657758261848));
#15037=CARTESIAN_POINT('Ctrl Pts',(-0.945943877838127,-0.30527573347708,
0.51387163140139));
#15038=CARTESIAN_POINT('Ctrl Pts',(-0.91968254693063,-0.29104845371857,
0.559515758398093));
#15039=CARTESIAN_POINT('Ctrl Pts',(-0.906170138993533,-0.28018331644634,
0.580957796077825));
#15040=CARTESIAN_POINT('Ctrl Pts',(-0.8813524085237,-0.254319232363049,
0.617994461173994));
#15041=CARTESIAN_POINT('Ctrl Pts',(-0.868789784891799,-0.237895043532788,
0.635412538795143));
#15042=CARTESIAN_POINT('Ctrl Pts',(-0.845715984518854,-0.199697230012983,
0.66581473268113));
#15043=CARTESIAN_POINT('Ctrl Pts',(-0.835214876415962,-0.177924977804098,
0.678808213394124));
#15044=CARTESIAN_POINT('Ctrl Pts',(-0.815669690204649,-0.124911173756694,
0.702247233627224));
#15045=CARTESIAN_POINT('Ctrl Pts',(-0.807662468433796,-0.0925528133349865,
0.711269279199861));
#15046=CARTESIAN_POINT('Ctrl Pts',(-0.803348093619616,-0.05953,0.716109245731214));
#15047=CARTESIAN_POINT('Origin',(-0.991065754692661,-0.05953,0.477272113029314));
#15048=CARTESIAN_POINT('Origin',(0.,-0.05953,0.));
#15049=CARTESIAN_POINT('',(-1.076188,-0.05953,1.31795018948079E-16));
#15050=CARTESIAN_POINT('Origin',(0.,-0.05953,0.));
#15051=CARTESIAN_POINT('',(-1.06075609691358,-0.05953,-0.181596019242328));
#15052=CARTESIAN_POINT('Origin',(0.,-0.05953,0.));
#15053=CARTESIAN_POINT('Origin',(-0.991065754692661,-0.05953,-0.477272113029314));
#15054=CARTESIAN_POINT('Origin',(-0.991065754692661,0.,-0.477272113029314));
#15055=CARTESIAN_POINT('',(-0.803348093619616,-0.05953,-0.716109245731215));
#15056=CARTESIAN_POINT('Ctrl Pts',(-0.803348093619616,-0.05953,-0.716109245731215));
#15057=CARTESIAN_POINT('Ctrl Pts',(-0.807662468433795,-0.0925528133349865,
-0.711269279199862));
#15058=CARTESIAN_POINT('Ctrl Pts',(-0.815669690204649,-0.124911173756694,
-0.702247233627224));
#15059=CARTESIAN_POINT('Ctrl Pts',(-0.835214876415962,-0.177924977804098,
-0.678808213394124));
#15060=CARTESIAN_POINT('Ctrl Pts',(-0.845715984518854,-0.199697230012983,
-0.66581473268113));
#15061=CARTESIAN_POINT('Ctrl Pts',(-0.868789784891799,-0.237895043532788,
-0.635412538795143));
#15062=CARTESIAN_POINT('Ctrl Pts',(-0.8813524085237,-0.254319232363049,
-0.617994461173994));
#15063=CARTESIAN_POINT('Ctrl Pts',(-0.906170138993533,-0.28018331644634,
-0.580957796077826));
#15064=CARTESIAN_POINT('Ctrl Pts',(-0.91968254693063,-0.29104845371857,
-0.559515758398093));
#15065=CARTESIAN_POINT('Ctrl Pts',(-0.945943877838127,-0.30527573347708,
-0.51387163140139));
#15066=CARTESIAN_POINT('Ctrl Pts',(-0.958671816228589,-0.308638795020976,
-0.489657758261848));
#15067=CARTESIAN_POINT('Ctrl Pts',(-0.980551951791748,-0.308638795020976,
-0.444223188605045));
#15068=CARTESIAN_POINT('Ctrl Pts',(-0.99154738033959,-0.30527573347708,
-0.419174982698463));
#15069=CARTESIAN_POINT('Ctrl Pts',(-1.01085972381132,-0.29104845371857,
-0.370184399726282));
#15070=CARTESIAN_POINT('Ctrl Pts',(-1.01919893537026,-0.28018331644634,
-0.346251081972725));
#15071=CARTESIAN_POINT('Ctrl Pts',(-1.03268176429485,-0.254319232363049,
-0.303755815985685));
#15072=CARTESIAN_POINT('Ctrl Pts',(-1.03846709802406,-0.237895043532788,
-0.283073967563097));
#15073=CARTESIAN_POINT('Ctrl Pts',(-1.04785021111757,-0.199697230012983,
-0.246078686169302));
#15074=CARTESIAN_POINT('Ctrl Pts',(-1.05146158959546,-0.177924977804098,
-0.229767286538461));
#15075=CARTESIAN_POINT('Ctrl Pts',(-1.05760072925372,-0.124911173756694,
-0.199872254546858));
#15076=CARTESIAN_POINT('Ctrl Pts',(-1.05966202740332,-0.0925528133349864,
-0.187986803072857));
#15077=CARTESIAN_POINT('Ctrl Pts',(-1.06075609691358,-0.05953,-0.181596019242328));
#15078=CARTESIAN_POINT('Origin',(-0.991065754692661,-0.05953,-0.477272113029314));
#15079=CARTESIAN_POINT('Origin',(0.,-0.05953,0.));
#15080=CARTESIAN_POINT('',(-0.519393123750572,-0.05953,-0.942555777842682));
#15081=CARTESIAN_POINT('Origin',(0.,-0.05953,0.));
#15082=CARTESIAN_POINT('Origin',(-0.244773027351946,-0.05953,-1.07242070340001));
#15083=CARTESIAN_POINT('Origin',(-0.244773027351946,0.,-1.07242070340001));
#15084=CARTESIAN_POINT('',(0.0589974094846125,-0.05953,-1.07456964270265));
#15085=CARTESIAN_POINT('Ctrl Pts',(0.0589974094846127,-0.05953,-1.07456964270265));
#15086=CARTESIAN_POINT('Ctrl Pts',(0.0525234025782722,-0.0925528133349865,
-1.07492508698591));
#15087=CARTESIAN_POINT('Ctrl Pts',(0.0404772621979744,-0.124911173756694,
-1.07556023164702));
#15088=CARTESIAN_POINT('Ctrl Pts',(0.0099656739833481,-0.177924977804098,
-1.07622728347683));
#15089=CARTESIAN_POINT('Ctrl Pts',(-0.00674037211528096,-0.199697230012983,
-1.07633607767727));
#15090=CARTESIAN_POINT('Ctrl Pts',(-0.044896043654098,-0.237895043532788,
-1.07542044338697));
#15091=CARTESIAN_POINT('Ctrl Pts',(-0.0663467128214644,-0.254319232363049,
-1.07438230428002));
#15092=CARTESIAN_POINT('Ctrl Pts',(-0.110776745452493,-0.28018331644634,
-1.07069360430242));
#15093=CARTESIAN_POINT('Ctrl Pts',(-0.135965654106109,-0.29104845371857,
-1.06788913840721));
#15094=CARTESIAN_POINT('Ctrl Pts',(-0.188025341585962,-0.30527573347708,
-1.05996242598502));
#15095=CARTESIAN_POINT('Ctrl Pts',(-0.214892249704082,-0.308638795020976,
-1.05481642595959));
#15096=CARTESIAN_POINT('Ctrl Pts',(-0.264056468041074,-0.308638795020976,
-1.04359501395068));
#15097=CARTESIAN_POINT('Ctrl Pts',(-0.290495481564827,-0.30527573347708,
-1.036574285215));
#15098=CARTESIAN_POINT('Ctrl Pts',(-0.340838910881557,-0.291048453718569,
-1.02112815447116));
#15099=CARTESIAN_POINT('Ctrl Pts',(-0.364750145543744,-0.28018331644634,
-1.01272583306292));
#15100=CARTESIAN_POINT('Ctrl Pts',(-0.406380688682952,-0.254319232363049,
-0.996771768218699));
#15101=CARTESIAN_POINT('Ctrl Pts',(-0.426157505475872,-0.237895043532788,
-0.988400002689705));
#15102=CARTESIAN_POINT('Ctrl Pts',(-0.460931856495794,-0.199697230012983,
-0.972669835243841));
#15103=CARTESIAN_POINT('Ctrl Pts',(-0.475936279901919,-0.177924977804098,
-0.965323333309091));
#15104=CARTESIAN_POINT('Ctrl Pts',(-0.503136848051454,-0.124911173756694,
-0.951483858396181));
#15105=CARTESIAN_POINT('Ctrl Pts',(-0.513714466572041,-0.0925528133349865,
-0.945684988399766));
#15106=CARTESIAN_POINT('Ctrl Pts',(-0.519393123750572,-0.05953,-0.942555777842682));
#15107=CARTESIAN_POINT('Origin',(-0.244773027351946,-0.05953,-1.07242070340001));
#15108=CARTESIAN_POINT('Origin',(0.,-0.05953,0.));
#15109=CARTESIAN_POINT('',(0.413083465285518,-0.05953,-0.993751811093549));
#15110=CARTESIAN_POINT('Origin',(0.,-0.05953,0.));
#15111=CARTESIAN_POINT('Origin',(0.685838782044607,-0.05953,-0.860014630714833));
#15112=CARTESIAN_POINT('Origin',(0.685838782044607,0.,-0.860014630714833));
#15113=CARTESIAN_POINT('',(0.876916659919095,-0.05953,-0.623857181492959));
#15114=CARTESIAN_POINT('Ctrl Pts',(0.876916659919095,-0.05953,-0.623857181492958));
#15115=CARTESIAN_POINT('Ctrl Pts',(0.873158080166742,-0.0925528133349865,
-0.62914037979579));
#15116=CARTESIAN_POINT('Ctrl Pts',(0.866144010579847,-0.124911173756694,
-0.638954437806245));
#15117=CARTESIAN_POINT('Ctrl Pts',(0.847641868610495,-0.177924977804098,
-0.663225258065736));
#15118=CARTESIAN_POINT('Ctrl Pts',(0.837310877969633,-0.199697230012983,
-0.676354402927683));
#15119=CARTESIAN_POINT('Ctrl Pts',(0.81280533416753,-0.237895043532788,
-0.705614819529209));
#15120=CARTESIAN_POINT('Ctrl Pts',(0.798619410861634,-0.254319232363049,
-0.721738358858166));
#15121=CARTESIAN_POINT('Ctrl Pts',(0.768033796848072,-0.28018331644634,
-0.754175290318038));
#15122=CARTESIAN_POINT('Ctrl Pts',(0.750136149454208,-0.29104845371857,
-0.772120216227122));
#15123=CARTESIAN_POINT('Ctrl Pts',(0.711480111898423,-0.30527573347708,
-0.807879894508811));
#15124=CARTESIAN_POINT('Ctrl Pts',(0.690705563850638,-0.308638795020976,
-0.825676810575913));
#15125=CARTESIAN_POINT('Ctrl Pts',(0.651278921914856,-0.308638795020976,
-0.857118508332695));
#15126=CARTESIAN_POINT('Ctrl Pts',(0.629305439856167,-0.30527573347708,
-0.873412008702649));
#15127=CARTESIAN_POINT('Ctrl Pts',(0.585840553788742,-0.29104845371857,
-0.903141581680914));
#15128=CARTESIAN_POINT('Ctrl Pts',(0.564362943424239,-0.28018331644634,
-0.916597376014514));
#15129=CARTESIAN_POINT('Ctrl Pts',(0.525933334162556,-0.254319232363049,
-0.939198248544427));
#15130=CARTESIAN_POINT('Ctrl Pts',(0.507057380724533,-0.237895043532788,
-0.949440676105255));
#15131=CARTESIAN_POINT('Ctrl Pts',(0.473077587363686,-0.199697230012983,
-0.966820759530997));
#15132=CARTESIAN_POINT('Ctrl Pts',(0.457978755888596,-0.177924977804098,
-0.973971221090534));
#15133=CARTESIAN_POINT('Ctrl Pts',(0.430199341854858,-0.124911173756694,
-0.986608710139579));
#15134=CARTESIAN_POINT('Ctrl Pts',(0.419070565453384,-0.0925528133349865,
-0.991263089003441));
#15135=CARTESIAN_POINT('Ctrl Pts',(0.413083465285518,-0.05953,-0.993751811093549));
#15136=CARTESIAN_POINT('Origin',(0.685838782044607,-0.05953,-0.860014630714833));
#15137=CARTESIAN_POINT('Origin',(0.,-0.208355,0.));
#15138=CARTESIAN_POINT('',(-1.076188,-0.35718,1.31795018948079E-16));
#15139=CARTESIAN_POINT('Origin',(0.,-0.35718,0.));
#15140=CARTESIAN_POINT('',(-1.076188,-0.208355,1.31795018948079E-16));
#15141=CARTESIAN_POINT('',(1.03449977959455,-0.05953,0.296632461748266));
#15142=CARTESIAN_POINT('Origin',(0.,-0.05953,0.));
#15143=CARTESIAN_POINT('',(1.03449977959455,-0.05953,-0.296632461748266));
#15144=CARTESIAN_POINT('Ctrl Pts',(1.03449977959455,-0.05953,0.296632461748267));
#15145=CARTESIAN_POINT('Ctrl Pts',(1.03628691421076,-0.0925528133349865,
0.290399865505497));
#15146=CARTESIAN_POINT('Ctrl Pts',(1.03958665287714,-0.124911173756694,
0.278797079997872));
#15147=CARTESIAN_POINT('Ctrl Pts',(1.0470264474309,-0.177924977804098,0.249198913998601));
#15148=CARTESIAN_POINT('Ctrl Pts',(1.05084995891418,-0.199697230012983,
0.232935932341942));
#15149=CARTESIAN_POINT('Ctrl Pts',(1.05844771715377,-0.237895043532788,
0.195533155353269));
#15150=CARTESIAN_POINT('Ctrl Pts',(1.06220882929878,-0.254319232363049,
0.17438929156337));
#15151=CARTESIAN_POINT('Ctrl Pts',(1.06849922508772,-0.28018331644634,0.130252399648131));
#15152=CARTESIAN_POINT('Ctrl Pts',(1.07137013248666,-0.29104845371857,0.105070977154072));
#15153=CARTESIAN_POINT('Ctrl Pts',(1.07522652957392,-0.30527573347708,0.0525526752791107));
#15154=CARTESIAN_POINT('Ctrl Pts',(1.076188,-0.308638795020976,0.025214283908933));
#15155=CARTESIAN_POINT('Ctrl Pts',(1.076188,-0.308638795020976,-0.025214283908933));
#15156=CARTESIAN_POINT('Ctrl Pts',(1.07522652957392,-0.30527573347708,-0.0525526752791107));
#15157=CARTESIAN_POINT('Ctrl Pts',(1.07137013248666,-0.29104845371857,-0.105070977154072));
#15158=CARTESIAN_POINT('Ctrl Pts',(1.06849922508772,-0.28018331644634,-0.130252399648131));
#15159=CARTESIAN_POINT('Ctrl Pts',(1.06220882929878,-0.254319232363049,
-0.17438929156337));
#15160=CARTESIAN_POINT('Ctrl Pts',(1.05844771715377,-0.237895043532788,
-0.195533155353269));
#15161=CARTESIAN_POINT('Ctrl Pts',(1.05084995891418,-0.199697230012983,
-0.232935932341942));
#15162=CARTESIAN_POINT('Ctrl Pts',(1.0470264474309,-0.177924977804098,-0.249198913998601));
#15163=CARTESIAN_POINT('Ctrl Pts',(1.03958665287714,-0.124911173756694,
-0.278797079997872));
#15164=CARTESIAN_POINT('Ctrl Pts',(1.03628691421076,-0.0925528133349865,
-0.290399865505497));
#15165=CARTESIAN_POINT('Ctrl Pts',(1.03449977959455,-0.05953,-0.296632461748267));
#15166=CARTESIAN_POINT('Origin',(0.,-0.05953,0.));
#15167=CARTESIAN_POINT('Origin',(0.,-0.05953,0.));
#15168=CARTESIAN_POINT('Origin',(1.1,-0.05953,0.));
#15169=CARTESIAN_POINT('Origin',(1.1,0.,0.));
#15170=CARTESIAN_POINT('Origin',(1.1,-0.05953,0.));
#15171=CARTESIAN_POINT('Origin',(0.,-0.35718,0.));
#15172=CARTESIAN_POINT('Origin',(0.,-0.05953,0.));
#16722=UNCERTAINTY_MEASURE_WITH_UNIT(LENGTH_MEASURE(0.001),#16800,
'DISTANCE_ACCURACY_VALUE',
'Maximum model space distance between geometric entities at asserted c
onnectivities');
#16750=UNCERTAINTY_MEASURE_WITH_UNIT(LENGTH_MEASURE(0.001),#16800,
'DISTANCE_ACCURACY_VALUE',
'Maximum model space distance between geometric entities at asserted c
onnectivities');
#16771=(
GEOMETRIC_REPRESENTATION_CONTEXT(3)
GLOBAL_UNCERTAINTY_ASSIGNED_CONTEXT((#16722))
GLOBAL_UNIT_ASSIGNED_CONTEXT((#16800,#16802,#16803))
REPRESENTATION_CONTEXT('','3D')
);
#16799=(
GEOMETRIC_REPRESENTATION_CONTEXT(3)
GLOBAL_UNCERTAINTY_ASSIGNED_CONTEXT((#16750))
GLOBAL_UNIT_ASSIGNED_CONTEXT((#16800,#16802,#16803))
REPRESENTATION_CONTEXT('','3D')
);
#16800=(
LENGTH_UNIT()
NAMED_UNIT(*)
SI_UNIT(.CENTI.,.METRE.)
);
#16802=(
NAMED_UNIT(*)
PLANE_ANGLE_UNIT()
SI_UNIT($,.RADIAN.)
);
#16803=(
NAMED_UNIT(*)
SI_UNIT($,.STERADIAN.)
SOLID_ANGLE_UNIT()
);
#16824=SHAPE_DEFINITION_REPRESENTATION(#16872,#17033);
#16872=PRODUCT_DEFINITION_SHAPE('',$,#17082);
#17033=SHAPE_REPRESENTATION('',(#10010),#16771);
#17061=PRODUCT_DEFINITION_CONTEXT('part definition',#17207,'design');
#17082=PRODUCT_DEFINITION('Cage','Cage',#17130,#17061);
#17130=PRODUCT_DEFINITION_FORMATION('',$,#17229);
#17207=APPLICATION_CONTEXT(
'Core Data for Automotive Mechanical Design Process');
#17208=PRODUCT_CONTEXT('part definition',#17207,'mechanical');
#17229=PRODUCT('Cage','Cage','Cage',(#17208));
#17320=COLOUR_RGB('Grey',0.48,0.52,0.57);
#17321=FILL_AREA_STYLE_COLOUR('',#17320);
#17322=FILL_AREA_STYLE('',(#17321));
#17323=SURFACE_STYLE_FILL_AREA(#17322);
#17324=SURFACE_SIDE_STYLE('',(#17323));
#17325=SURFACE_STYLE_USAGE(.BOTH.,#17324);
#17326=PRESENTATION_STYLE_ASSIGNMENT((#17325));
ENDSEC;
END-ISO-10303-21;
